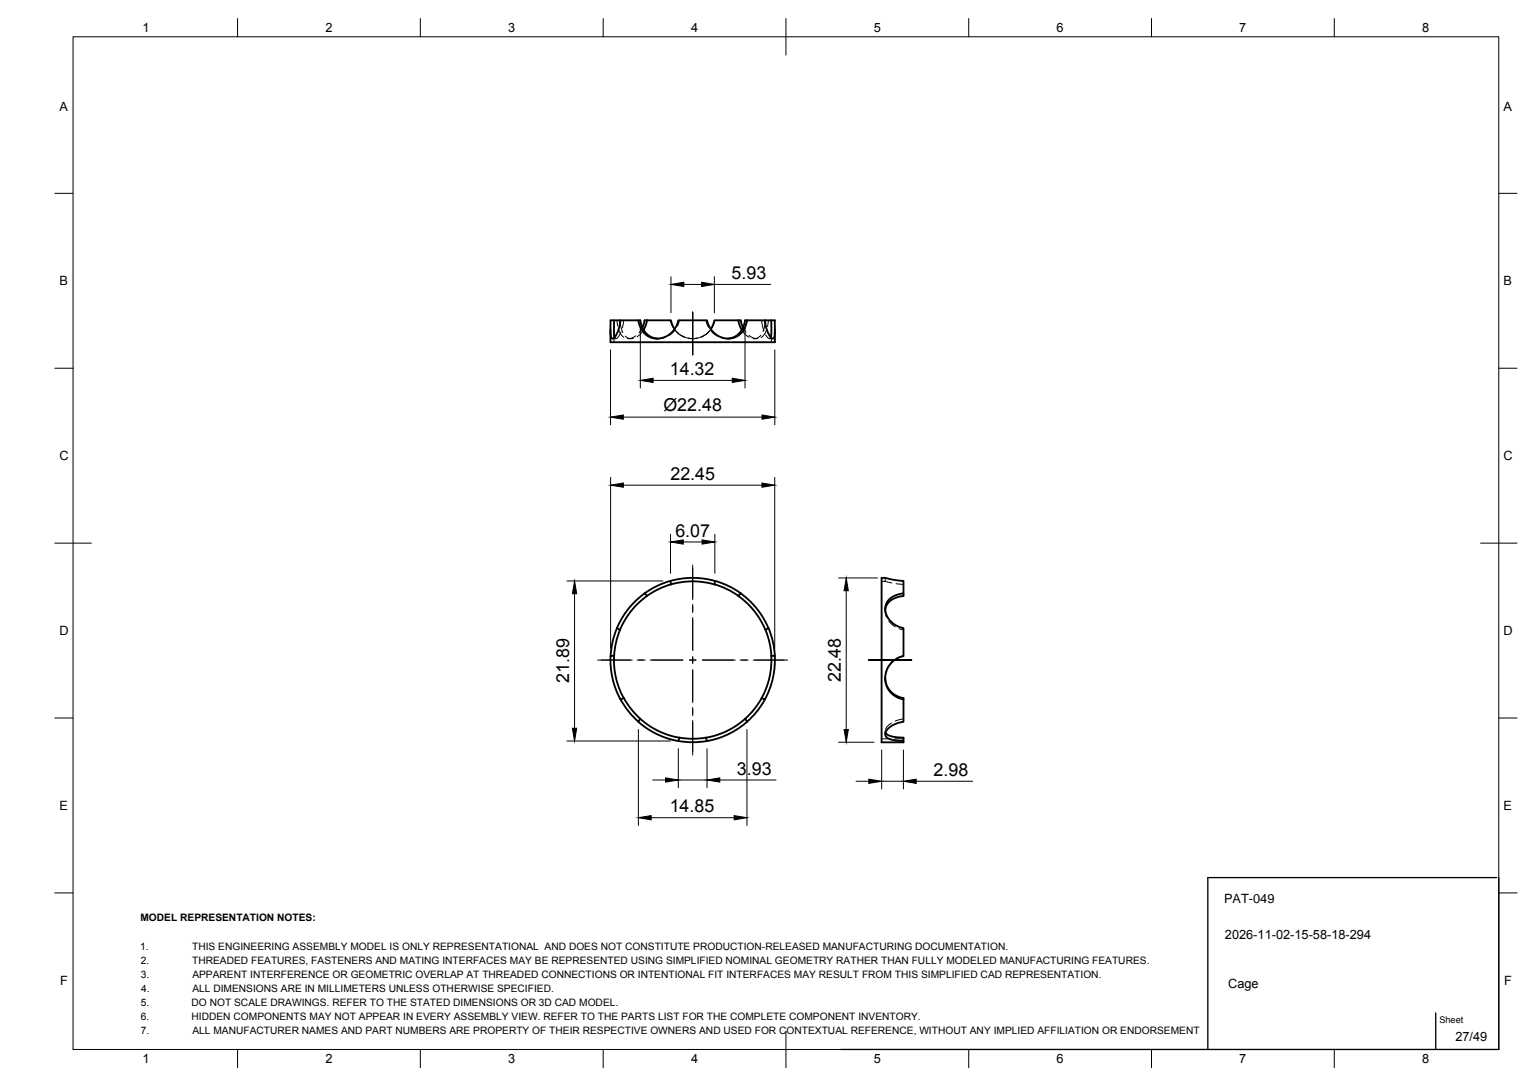
ISO-10303-21;
HEADER;
/* Generated by software containing ST-Developer
 * from STEP Tools, Inc. (www.steptools.com) 
 */

FILE_DESCRIPTION(
/* description */ ('Hand drill press frame (manual)'),
/* implementation_level */ '2;1');

FILE_NAME(
/* name */ 'Cage.step',
/* time_stamp */ '2026-10-28T03:25:28-07:00',
/* author */ (''),
/* organization */ (''),
/* preprocessor_version */ 'ST-DEVELOPER v20.2',
/* originating_system */ 'Autodesk Translation Framework v15.17.0.0',
/* authorisation */ '');

FILE_SCHEMA (('AUTOMOTIVE_DESIGN { 1 0 10303 214 3 1 1 }'));
ENDSEC;

DATA;
#10=MECHANICAL_DESIGN_GEOMETRIC_PRESENTATION_REPRESENTATION('',(#645),#33299);
#464=SPHERICAL_SURFACE('',#13660,0.309556);
#465=SPHERICAL_SURFACE('',#13676,0.309556);
#466=SPHERICAL_SURFACE('',#13681,0.309556);
#467=SPHERICAL_SURFACE('',#13687,0.309556);
#468=SPHERICAL_SURFACE('',#13692,0.309556);
#469=SPHERICAL_SURFACE('',#13697,0.309556);
#470=SPHERICAL_SURFACE('',#13705,0.309556);
#506=B_SPLINE_CURVE_WITH_KNOTS('',3,(#19268,#19269,#19270,#19271,#19272,
#19273,#19274,#19275,#19276,#19277,#19278,#19279,#19280,#19281,#19282,#19283,
#19284,#19285,#19286,#19287,#19288,#19289),.UNSPECIFIED.,.F.,.F.,(4,2,2,
2,2,2,2,2,2,2,4),(0.0591825211272536,0.157966726598481,0.236950089897721,
0.315933453196962,0.391576304923761,0.46721915665056,0.54286200837736,0.618504860104159,
0.697488223403399,0.77647158670264,0.875255792173867),.UNSPECIFIED.);
#507=B_SPLINE_CURVE_WITH_KNOTS('',3,(#19293,#19294,#19295,#19296,#19297,
#19298,#19299,#19300,#19301,#19302,#19303,#19304,#19305,#19306,#19307,#19308,
#19309,#19310,#19311,#19312,#19313,#19314),.UNSPECIFIED.,.F.,.F.,(4,2,2,
2,2,2,2,2,2,2,4),(0.0581119756758434,0.106553146291161,0.213106292582322,
0.30849933801665,0.386091982889075,0.4636846277615,0.541277272633925,0.61886991750635,
0.714262962940678,0.820816109231839,0.869257279847157),.UNSPECIFIED.);
#508=B_SPLINE_CURVE_WITH_KNOTS('',3,(#19320,#19321,#19322,#19323,#19324,
#19325,#19326,#19327,#19328,#19329,#19330,#19331,#19332,#19333,#19334,#19335,
#19336,#19337,#19338,#19339,#19340,#19341),.UNSPECIFIED.,.F.,.F.,(4,2,2,
2,2,2,2,2,2,2,4),(0.0581119756758434,0.106553146291161,0.213106292582322,
0.30849933801665,0.386091982889075,0.4636846277615,0.541277272633925,0.61886991750635,
0.714262962940679,0.820816109231839,0.869257279847157),.UNSPECIFIED.);
#509=B_SPLINE_CURVE_WITH_KNOTS('',3,(#19345,#19346,#19347,#19348,#19349,
#19350,#19351,#19352,#19353,#19354,#19355,#19356,#19357,#19358,#19359,#19360,
#19361,#19362,#19363,#19364,#19365,#19366),.UNSPECIFIED.,.F.,.F.,(4,2,2,
2,2,2,2,2,2,2,4),(0.0581119756758433,0.106553146291161,0.213106292582322,
0.308499338016649,0.386091982889075,0.4636846277615,0.541277272633925,0.61886991750635,
0.714262962940678,0.820816109231839,0.869257279847157),.UNSPECIFIED.);
#510=B_SPLINE_CURVE_WITH_KNOTS('',3,(#19375,#19376,#19377,#19378,#19379,
#19380,#19381,#19382,#19383,#19384,#19385,#19386,#19387,#19388,#19389,#19390,
#19391,#19392,#19393,#19394,#19395,#19396),.UNSPECIFIED.,.F.,.F.,(4,2,2,
2,2,2,2,2,2,2,4),(0.0581119756758433,0.106553146291161,0.213106292582322,
0.30849933801665,0.386091982889075,0.4636846277615,0.541277272633925,0.61886991750635,
0.714262962940678,0.820816109231839,0.869257279847157),.UNSPECIFIED.);
#511=B_SPLINE_CURVE_WITH_KNOTS('',3,(#19400,#19401,#19402,#19403,#19404,
#19405,#19406,#19407,#19408,#19409,#19410,#19411,#19412,#19413,#19414,#19415,
#19416,#19417,#19418,#19419,#19420,#19421),.UNSPECIFIED.,.F.,.F.,(4,2,2,
2,2,2,2,2,2,2,4),(0.0581119756758434,0.106553146291161,0.213106292582322,
0.30849933801665,0.386091982889075,0.4636846277615,0.541277272633925,0.61886991750635,
0.714262962940678,0.820816109231839,0.869257279847157),.UNSPECIFIED.);
#512=B_SPLINE_CURVE_WITH_KNOTS('',3,(#19425,#19426,#19427,#19428,#19429,
#19430,#19431,#19432,#19433,#19434,#19435,#19436,#19437,#19438,#19439,#19440,
#19441,#19442,#19443,#19444,#19445,#19446),.UNSPECIFIED.,.F.,.F.,(4,2,2,
2,2,2,2,2,2,2,4),(0.0581119756758434,0.106553146291161,0.213106292582322,
0.30849933801665,0.386091982889075,0.4636846277615,0.541277272633925,0.61886991750635,
0.714262962940678,0.820816109231839,0.869257279847157),.UNSPECIFIED.);
#513=B_SPLINE_CURVE_WITH_KNOTS('',3,(#19450,#19451,#19452,#19453,#19454,
#19455,#19456,#19457,#19458,#19459,#19460,#19461,#19462,#19463,#19464,#19465,
#19466,#19467,#19468,#19469,#19470,#19471),.UNSPECIFIED.,.F.,.F.,(4,2,2,
2,2,2,2,2,2,2,4),(0.0581119756758433,0.106553146291161,0.213106292582322,
0.30849933801665,0.386091982889075,0.4636846277615,0.541277272633925,0.61886991750635,
0.714262962940678,0.820816109231839,0.869257279847157),.UNSPECIFIED.);
#514=B_SPLINE_CURVE_WITH_KNOTS('',3,(#19479,#19480,#19481,#19482,#19483,
#19484,#19485,#19486,#19487,#19488,#19489,#19490,#19491,#19492,#19493,#19494,
#19495,#19496,#19497,#19498,#19499,#19500),.UNSPECIFIED.,.F.,.F.,(4,2,2,
2,2,2,2,2,2,2,4),(0.0591825211272536,0.157966726598481,0.236950089897721,
0.315933453196962,0.391576304923761,0.467219156650561,0.54286200837736,
0.618504860104159,0.697488223403399,0.77647158670264,0.875255792173867),
 .UNSPECIFIED.);
#515=B_SPLINE_CURVE_WITH_KNOTS('',3,(#19508,#19509,#19510,#19511,#19512,
#19513,#19514,#19515,#19516,#19517,#19518,#19519,#19520,#19521,#19522,#19523,
#19524,#19525,#19526,#19527,#19528,#19529),.UNSPECIFIED.,.F.,.F.,(4,2,2,
2,2,2,2,2,2,2,4),(0.0591825211272536,0.157966726598481,0.236950089897722,
0.315933453196962,0.391576304923761,0.467219156650561,0.54286200837736,
0.618504860104159,0.697488223403399,0.77647158670264,0.875255792173867),
 .UNSPECIFIED.);
#516=B_SPLINE_CURVE_WITH_KNOTS('',3,(#19539,#19540,#19541,#19542,#19543,
#19544,#19545,#19546,#19547,#19548,#19549,#19550,#19551,#19552,#19553,#19554,
#19555,#19556,#19557,#19558,#19559,#19560),.UNSPECIFIED.,.F.,.F.,(4,2,2,
2,2,2,2,2,2,2,4),(0.0591825211272536,0.157966726598481,0.236950089897721,
0.315933453196962,0.391576304923761,0.46721915665056,0.54286200837736,0.618504860104159,
0.697488223403399,0.77647158670264,0.875255792173867),.UNSPECIFIED.);
#517=B_SPLINE_CURVE_WITH_KNOTS('',3,(#19568,#19569,#19570,#19571,#19572,
#19573,#19574,#19575,#19576,#19577,#19578,#19579,#19580,#19581,#19582,#19583,
#19584,#19585,#19586,#19587,#19588,#19589),.UNSPECIFIED.,.F.,.F.,(4,2,2,
2,2,2,2,2,2,2,4),(0.0591825211272536,0.157966726598481,0.236950089897721,
0.315933453196962,0.391576304923761,0.46721915665056,0.542862008377359,
0.618504860104159,0.697488223403399,0.776471586702639,0.875255792173867),
 .UNSPECIFIED.);
#518=B_SPLINE_CURVE_WITH_KNOTS('',3,(#19597,#19598,#19599,#19600,#19601,
#19602,#19603,#19604,#19605,#19606,#19607,#19608,#19609,#19610,#19611,#19612,
#19613,#19614,#19615,#19616,#19617,#19618),.UNSPECIFIED.,.F.,.F.,(4,2,2,
2,2,2,2,2,2,2,4),(0.0591825211272536,0.157966726598481,0.236950089897721,
0.315933453196962,0.391576304923761,0.46721915665056,0.54286200837736,0.618504860104159,
0.697488223403399,0.77647158670264,0.875255792173867),.UNSPECIFIED.);
#519=B_SPLINE_CURVE_WITH_KNOTS('',3,(#19627,#19628,#19629,#19630,#19631,
#19632,#19633,#19634,#19635,#19636,#19637,#19638,#19639,#19640,#19641,#19642,
#19643,#19644,#19645,#19646,#19647,#19648),.UNSPECIFIED.,.F.,.F.,(4,2,2,
2,2,2,2,2,2,2,4),(0.0591825211272536,0.157966726598481,0.236950089897721,
0.315933453196962,0.391576304923761,0.46721915665056,0.542862008377359,
0.618504860104159,0.697488223403399,0.776471586702639,0.875255792173867),
 .UNSPECIFIED.);
#549=SHAPE_REPRESENTATION_RELATIONSHIP('SRR','None',#33509,#594);
#594=ADVANCED_BREP_SHAPE_REPRESENTATION('',(#697),#33271);
#645=STYLED_ITEM('',(#33814),#697);
#697=MANIFOLD_SOLID_BREP('Continuous crown cage',#12663);
#840=FACE_BOUND('',#2404,.T.);
#1021=PLANE('',#13673);
#1022=PLANE('',#13678);
#1023=PLANE('',#13683);
#1024=PLANE('',#13689);
#1025=PLANE('',#13694);
#1026=PLANE('',#13703);
#1027=PLANE('',#13707);
#1028=PLANE('',#13708);
#1579=FACE_OUTER_BOUND('',#2388,.T.);
#1580=FACE_OUTER_BOUND('',#2389,.T.);
#1581=FACE_OUTER_BOUND('',#2390,.T.);
#1582=FACE_OUTER_BOUND('',#2391,.T.);
#1583=FACE_OUTER_BOUND('',#2392,.T.);
#1584=FACE_OUTER_BOUND('',#2393,.T.);
#1585=FACE_OUTER_BOUND('',#2394,.T.);
#1586=FACE_OUTER_BOUND('',#2395,.T.);
#1587=FACE_OUTER_BOUND('',#2396,.T.);
#1588=FACE_OUTER_BOUND('',#2397,.T.);
#1589=FACE_OUTER_BOUND('',#2398,.T.);
#1590=FACE_OUTER_BOUND('',#2399,.T.);
#1591=FACE_OUTER_BOUND('',#2400,.T.);
#1592=FACE_OUTER_BOUND('',#2401,.T.);
#1593=FACE_OUTER_BOUND('',#2402,.T.);
#1594=FACE_OUTER_BOUND('',#2403,.T.);
#1595=FACE_OUTER_BOUND('',#2405,.T.);
#2388=EDGE_LOOP('',(#9525,#9526,#9527,#9528));
#2389=EDGE_LOOP('',(#9529,#9530,#9531,#9532,#9533,#9534,#9535,#9536,#9537,
#9538,#9539,#9540,#9541,#9542,#9543,#9544,#9545,#9546));
#2390=EDGE_LOOP('',(#9547,#9548,#9549,#9550));
#2391=EDGE_LOOP('',(#9551,#9552,#9553,#9554));
#2392=EDGE_LOOP('',(#9555,#9556,#9557,#9558));
#2393=EDGE_LOOP('',(#9559,#9560,#9561,#9562));
#2394=EDGE_LOOP('',(#9563,#9564,#9565,#9566,#9567,#9568));
#2395=EDGE_LOOP('',(#9569,#9570,#9571,#9572));
#2396=EDGE_LOOP('',(#9573,#9574,#9575,#9576));
#2397=EDGE_LOOP('',(#9577,#9578,#9579,#9580));
#2398=EDGE_LOOP('',(#9581,#9582,#9583,#9584));
#2399=EDGE_LOOP('',(#9585,#9586,#9587,#9588));
#2400=EDGE_LOOP('',(#9589,#9590,#9591,#9592,#9593,#9594,#9595,#9596,#9597,
#9598,#9599,#9600,#9601,#9602,#9603,#9604,#9605,#9606));
#2401=EDGE_LOOP('',(#9607,#9608,#9609,#9610));
#2402=EDGE_LOOP('',(#9611,#9612,#9613,#9614));
#2403=EDGE_LOOP('',(#9615));
#2404=EDGE_LOOP('',(#9616));
#2405=EDGE_LOOP('',(#9617,#9618,#9619,#9620));
#3213=LINE('',#19370,#4378);
#3214=LINE('',#19623,#4379);
#4378=VECTOR('',#15654,1.123812);
#4379=VECTOR('',#15723,1.076188);
#5422=CIRCLE('',#13661,0.303778037777585);
#5423=CIRCLE('',#13662,0.303778037777585);
#5424=CIRCLE('',#13664,1.123812);
#5425=CIRCLE('',#13665,1.123812);
#5426=CIRCLE('',#13666,1.123812);
#5427=CIRCLE('',#13667,1.123812);
#5428=CIRCLE('',#13668,1.123812);
#5429=CIRCLE('',#13669,1.123812);
#5430=CIRCLE('',#13670,1.123812);
#5431=CIRCLE('',#13671,1.123812);
#5432=CIRCLE('',#13672,1.123812);
#5433=CIRCLE('',#13674,1.076188);
#5434=CIRCLE('',#13675,0.303778037777585);
#5435=CIRCLE('',#13677,0.303778037777585);
#5436=CIRCLE('',#13679,1.076188);
#5437=CIRCLE('',#13680,0.303778037777585);
#5438=CIRCLE('',#13682,0.303778037777585);
#5439=CIRCLE('',#13684,1.076188);
#5440=CIRCLE('',#13685,1.076188);
#5441=CIRCLE('',#13686,0.303778037777585);
#5442=CIRCLE('',#13688,0.303778037777585);
#5443=CIRCLE('',#13690,1.076188);
#5444=CIRCLE('',#13691,0.303778037777585);
#5445=CIRCLE('',#13693,0.303778037777585);
#5446=CIRCLE('',#13695,1.076188);
#5447=CIRCLE('',#13696,0.303778037777585);
#5448=CIRCLE('',#13698,0.303778037777585);
#5449=CIRCLE('',#13700,1.076188);
#5450=CIRCLE('',#13701,1.076188);
#5451=CIRCLE('',#13702,1.076188);
#5452=CIRCLE('',#13704,0.303778037777585);
#5453=CIRCLE('',#13706,0.303778037777585);
#5989=VERTEX_POINT('',#19266);
#5990=VERTEX_POINT('',#19267);
#5991=VERTEX_POINT('',#19290);
#5992=VERTEX_POINT('',#19292);
#5993=VERTEX_POINT('',#19317);
#5994=VERTEX_POINT('',#19319);
#5995=VERTEX_POINT('',#19342);
#5996=VERTEX_POINT('',#19344);
#5997=VERTEX_POINT('',#19367);
#5998=VERTEX_POINT('',#19369);
#5999=VERTEX_POINT('',#19372);
#6000=VERTEX_POINT('',#19374);
#6001=VERTEX_POINT('',#19397);
#6002=VERTEX_POINT('',#19399);
#6003=VERTEX_POINT('',#19422);
#6004=VERTEX_POINT('',#19424);
#6005=VERTEX_POINT('',#19447);
#6006=VERTEX_POINT('',#19449);
#6007=VERTEX_POINT('',#19474);
#6008=VERTEX_POINT('',#19478);
#6009=VERTEX_POINT('',#19503);
#6010=VERTEX_POINT('',#19507);
#6011=VERTEX_POINT('',#19532);
#6012=VERTEX_POINT('',#19534);
#6013=VERTEX_POINT('',#19538);
#6014=VERTEX_POINT('',#19563);
#6015=VERTEX_POINT('',#19567);
#6016=VERTEX_POINT('',#19592);
#6017=VERTEX_POINT('',#19596);
#6018=VERTEX_POINT('',#19621);
#6019=VERTEX_POINT('',#19624);
#6020=VERTEX_POINT('',#19626);
#7291=EDGE_CURVE('',#5989,#5990,#506,.T.);
#7292=EDGE_CURVE('',#5991,#5989,#5422,.T.);
#7293=EDGE_CURVE('',#5992,#5991,#507,.T.);
#7294=EDGE_CURVE('',#5990,#5992,#5423,.T.);
#7295=EDGE_CURVE('',#5993,#5991,#5424,.T.);
#7296=EDGE_CURVE('',#5993,#5994,#508,.T.);
#7297=EDGE_CURVE('',#5995,#5994,#5425,.T.);
#7298=EDGE_CURVE('',#5995,#5996,#509,.T.);
#7299=EDGE_CURVE('',#5997,#5996,#5426,.T.);
#7300=EDGE_CURVE('',#5997,#5998,#3213,.T.);
#7301=EDGE_CURVE('',#5998,#5998,#5427,.T.);
#7302=EDGE_CURVE('',#5999,#5997,#5428,.T.);
#7303=EDGE_CURVE('',#5999,#6000,#510,.T.);
#7304=EDGE_CURVE('',#6001,#6000,#5429,.T.);
#7305=EDGE_CURVE('',#6001,#6002,#511,.T.);
#7306=EDGE_CURVE('',#6003,#6002,#5430,.T.);
#7307=EDGE_CURVE('',#6003,#6004,#512,.T.);
#7308=EDGE_CURVE('',#6005,#6004,#5431,.T.);
#7309=EDGE_CURVE('',#6005,#6006,#513,.T.);
#7310=EDGE_CURVE('',#5992,#6006,#5432,.T.);
#7311=EDGE_CURVE('',#5989,#6007,#5433,.T.);
#7312=EDGE_CURVE('',#6007,#5993,#5434,.T.);
#7313=EDGE_CURVE('',#6008,#6007,#514,.T.);
#7314=EDGE_CURVE('',#5994,#6008,#5435,.T.);
#7315=EDGE_CURVE('',#6008,#6009,#5436,.T.);
#7316=EDGE_CURVE('',#6009,#5995,#5437,.T.);
#7317=EDGE_CURVE('',#6010,#6009,#515,.T.);
#7318=EDGE_CURVE('',#5996,#6010,#5438,.T.);
#7319=EDGE_CURVE('',#6010,#6011,#5439,.T.);
#7320=EDGE_CURVE('',#6011,#6012,#5440,.T.);
#7321=EDGE_CURVE('',#6012,#5999,#5441,.T.);
#7322=EDGE_CURVE('',#6013,#6012,#516,.T.);
#7323=EDGE_CURVE('',#6000,#6013,#5442,.T.);
#7324=EDGE_CURVE('',#6013,#6014,#5443,.T.);
#7325=EDGE_CURVE('',#6014,#6001,#5444,.T.);
#7326=EDGE_CURVE('',#6015,#6014,#517,.T.);
#7327=EDGE_CURVE('',#6002,#6015,#5445,.T.);
#7328=EDGE_CURVE('',#6015,#6016,#5446,.T.);
#7329=EDGE_CURVE('',#6016,#6003,#5447,.T.);
#7330=EDGE_CURVE('',#6017,#6016,#518,.T.);
#7331=EDGE_CURVE('',#6004,#6017,#5448,.T.);
#7332=EDGE_CURVE('',#6018,#6018,#5449,.T.);
#7333=EDGE_CURVE('',#6018,#6011,#3214,.T.);
#7334=EDGE_CURVE('',#6019,#5990,#5450,.T.);
#7335=EDGE_CURVE('',#6019,#6020,#519,.T.);
#7336=EDGE_CURVE('',#6017,#6020,#5451,.T.);
#7337=EDGE_CURVE('',#6006,#6019,#5452,.T.);
#7338=EDGE_CURVE('',#6020,#6005,#5453,.T.);
#9525=ORIENTED_EDGE('',*,*,#7291,.F.);
#9526=ORIENTED_EDGE('',*,*,#7292,.F.);
#9527=ORIENTED_EDGE('',*,*,#7293,.F.);
#9528=ORIENTED_EDGE('',*,*,#7294,.F.);
#9529=ORIENTED_EDGE('',*,*,#7293,.T.);
#9530=ORIENTED_EDGE('',*,*,#7295,.F.);
#9531=ORIENTED_EDGE('',*,*,#7296,.T.);
#9532=ORIENTED_EDGE('',*,*,#7297,.F.);
#9533=ORIENTED_EDGE('',*,*,#7298,.T.);
#9534=ORIENTED_EDGE('',*,*,#7299,.F.);
#9535=ORIENTED_EDGE('',*,*,#7300,.T.);
#9536=ORIENTED_EDGE('',*,*,#7301,.F.);
#9537=ORIENTED_EDGE('',*,*,#7300,.F.);
#9538=ORIENTED_EDGE('',*,*,#7302,.F.);
#9539=ORIENTED_EDGE('',*,*,#7303,.T.);
#9540=ORIENTED_EDGE('',*,*,#7304,.F.);
#9541=ORIENTED_EDGE('',*,*,#7305,.T.);
#9542=ORIENTED_EDGE('',*,*,#7306,.F.);
#9543=ORIENTED_EDGE('',*,*,#7307,.T.);
#9544=ORIENTED_EDGE('',*,*,#7308,.F.);
#9545=ORIENTED_EDGE('',*,*,#7309,.T.);
#9546=ORIENTED_EDGE('',*,*,#7310,.F.);
#9547=ORIENTED_EDGE('',*,*,#7292,.T.);
#9548=ORIENTED_EDGE('',*,*,#7311,.T.);
#9549=ORIENTED_EDGE('',*,*,#7312,.T.);
#9550=ORIENTED_EDGE('',*,*,#7295,.T.);
#9551=ORIENTED_EDGE('',*,*,#7313,.F.);
#9552=ORIENTED_EDGE('',*,*,#7314,.F.);
#9553=ORIENTED_EDGE('',*,*,#7296,.F.);
#9554=ORIENTED_EDGE('',*,*,#7312,.F.);
#9555=ORIENTED_EDGE('',*,*,#7314,.T.);
#9556=ORIENTED_EDGE('',*,*,#7315,.T.);
#9557=ORIENTED_EDGE('',*,*,#7316,.T.);
#9558=ORIENTED_EDGE('',*,*,#7297,.T.);
#9559=ORIENTED_EDGE('',*,*,#7317,.F.);
#9560=ORIENTED_EDGE('',*,*,#7318,.F.);
#9561=ORIENTED_EDGE('',*,*,#7298,.F.);
#9562=ORIENTED_EDGE('',*,*,#7316,.F.);
#9563=ORIENTED_EDGE('',*,*,#7318,.T.);
#9564=ORIENTED_EDGE('',*,*,#7319,.T.);
#9565=ORIENTED_EDGE('',*,*,#7320,.T.);
#9566=ORIENTED_EDGE('',*,*,#7321,.T.);
#9567=ORIENTED_EDGE('',*,*,#7302,.T.);
#9568=ORIENTED_EDGE('',*,*,#7299,.T.);
#9569=ORIENTED_EDGE('',*,*,#7322,.F.);
#9570=ORIENTED_EDGE('',*,*,#7323,.F.);
#9571=ORIENTED_EDGE('',*,*,#7303,.F.);
#9572=ORIENTED_EDGE('',*,*,#7321,.F.);
#9573=ORIENTED_EDGE('',*,*,#7323,.T.);
#9574=ORIENTED_EDGE('',*,*,#7324,.T.);
#9575=ORIENTED_EDGE('',*,*,#7325,.T.);
#9576=ORIENTED_EDGE('',*,*,#7304,.T.);
#9577=ORIENTED_EDGE('',*,*,#7326,.F.);
#9578=ORIENTED_EDGE('',*,*,#7327,.F.);
#9579=ORIENTED_EDGE('',*,*,#7305,.F.);
#9580=ORIENTED_EDGE('',*,*,#7325,.F.);
#9581=ORIENTED_EDGE('',*,*,#7327,.T.);
#9582=ORIENTED_EDGE('',*,*,#7328,.T.);
#9583=ORIENTED_EDGE('',*,*,#7329,.T.);
#9584=ORIENTED_EDGE('',*,*,#7306,.T.);
#9585=ORIENTED_EDGE('',*,*,#7307,.F.);
#9586=ORIENTED_EDGE('',*,*,#7329,.F.);
#9587=ORIENTED_EDGE('',*,*,#7330,.F.);
#9588=ORIENTED_EDGE('',*,*,#7331,.F.);
#9589=ORIENTED_EDGE('',*,*,#7332,.F.);
#9590=ORIENTED_EDGE('',*,*,#7333,.T.);
#9591=ORIENTED_EDGE('',*,*,#7319,.F.);
#9592=ORIENTED_EDGE('',*,*,#7317,.T.);
#9593=ORIENTED_EDGE('',*,*,#7315,.F.);
#9594=ORIENTED_EDGE('',*,*,#7313,.T.);
#9595=ORIENTED_EDGE('',*,*,#7311,.F.);
#9596=ORIENTED_EDGE('',*,*,#7291,.T.);
#9597=ORIENTED_EDGE('',*,*,#7334,.F.);
#9598=ORIENTED_EDGE('',*,*,#7335,.T.);
#9599=ORIENTED_EDGE('',*,*,#7336,.F.);
#9600=ORIENTED_EDGE('',*,*,#7330,.T.);
#9601=ORIENTED_EDGE('',*,*,#7328,.F.);
#9602=ORIENTED_EDGE('',*,*,#7326,.T.);
#9603=ORIENTED_EDGE('',*,*,#7324,.F.);
#9604=ORIENTED_EDGE('',*,*,#7322,.T.);
#9605=ORIENTED_EDGE('',*,*,#7320,.F.);
#9606=ORIENTED_EDGE('',*,*,#7333,.F.);
#9607=ORIENTED_EDGE('',*,*,#7294,.T.);
#9608=ORIENTED_EDGE('',*,*,#7310,.T.);
#9609=ORIENTED_EDGE('',*,*,#7337,.T.);
#9610=ORIENTED_EDGE('',*,*,#7334,.T.);
#9611=ORIENTED_EDGE('',*,*,#7309,.F.);
#9612=ORIENTED_EDGE('',*,*,#7338,.F.);
#9613=ORIENTED_EDGE('',*,*,#7335,.F.);
#9614=ORIENTED_EDGE('',*,*,#7337,.F.);
#9615=ORIENTED_EDGE('',*,*,#7301,.T.);
#9616=ORIENTED_EDGE('',*,*,#7332,.T.);
#9617=ORIENTED_EDGE('',*,*,#7331,.T.);
#9618=ORIENTED_EDGE('',*,*,#7336,.T.);
#9619=ORIENTED_EDGE('',*,*,#7338,.T.);
#9620=ORIENTED_EDGE('',*,*,#7308,.T.);
#11877=CYLINDRICAL_SURFACE('',#13663,1.123812);
#11878=CYLINDRICAL_SURFACE('',#13699,1.076188);
#12188=ADVANCED_FACE('',(#1579),#464,.F.);
#12189=ADVANCED_FACE('',(#1580),#11877,.T.);
#12190=ADVANCED_FACE('',(#1581),#1021,.T.);
#12191=ADVANCED_FACE('',(#1582),#465,.F.);
#12192=ADVANCED_FACE('',(#1583),#1022,.T.);
#12193=ADVANCED_FACE('',(#1584),#466,.F.);
#12194=ADVANCED_FACE('',(#1585),#1023,.T.);
#12195=ADVANCED_FACE('',(#1586),#467,.F.);
#12196=ADVANCED_FACE('',(#1587),#1024,.T.);
#12197=ADVANCED_FACE('',(#1588),#468,.F.);
#12198=ADVANCED_FACE('',(#1589),#1025,.T.);
#12199=ADVANCED_FACE('',(#1590),#469,.F.);
#12200=ADVANCED_FACE('',(#1591),#11878,.F.);
#12201=ADVANCED_FACE('',(#1592),#1026,.T.);
#12202=ADVANCED_FACE('',(#1593),#470,.F.);
#12203=ADVANCED_FACE('',(#1594,#840),#1027,.T.);
#12204=ADVANCED_FACE('',(#1595),#1028,.T.);
#12663=CLOSED_SHELL('',(#12188,#12189,#12190,#12191,#12192,#12193,#12194,
#12195,#12196,#12197,#12198,#12199,#12200,#12201,#12202,#12203,#12204));
#13659=AXIS2_PLACEMENT_3D('',#19264,#15638,#15639);
#13660=AXIS2_PLACEMENT_3D('',#19265,#15640,#15641);
#13661=AXIS2_PLACEMENT_3D('',#19291,#15642,#15643);
#13662=AXIS2_PLACEMENT_3D('',#19315,#15644,#15645);
#13663=AXIS2_PLACEMENT_3D('',#19316,#15646,#15647);
#13664=AXIS2_PLACEMENT_3D('',#19318,#15648,#15649);
#13665=AXIS2_PLACEMENT_3D('',#19343,#15650,#15651);
#13666=AXIS2_PLACEMENT_3D('',#19368,#15652,#15653);
#13667=AXIS2_PLACEMENT_3D('',#19371,#15655,#15656);
#13668=AXIS2_PLACEMENT_3D('',#19373,#15657,#15658);
#13669=AXIS2_PLACEMENT_3D('',#19398,#15659,#15660);
#13670=AXIS2_PLACEMENT_3D('',#19423,#15661,#15662);
#13671=AXIS2_PLACEMENT_3D('',#19448,#15663,#15664);
#13672=AXIS2_PLACEMENT_3D('',#19472,#15665,#15666);
#13673=AXIS2_PLACEMENT_3D('',#19473,#15667,#15668);
#13674=AXIS2_PLACEMENT_3D('',#19475,#15669,#15670);
#13675=AXIS2_PLACEMENT_3D('',#19476,#15671,#15672);
#13676=AXIS2_PLACEMENT_3D('',#19477,#15673,#15674);
#13677=AXIS2_PLACEMENT_3D('',#19501,#15675,#15676);
#13678=AXIS2_PLACEMENT_3D('',#19502,#15677,#15678);
#13679=AXIS2_PLACEMENT_3D('',#19504,#15679,#15680);
#13680=AXIS2_PLACEMENT_3D('',#19505,#15681,#15682);
#13681=AXIS2_PLACEMENT_3D('',#19506,#15683,#15684);
#13682=AXIS2_PLACEMENT_3D('',#19530,#15685,#15686);
#13683=AXIS2_PLACEMENT_3D('',#19531,#15687,#15688);
#13684=AXIS2_PLACEMENT_3D('',#19533,#15689,#15690);
#13685=AXIS2_PLACEMENT_3D('',#19535,#15691,#15692);
#13686=AXIS2_PLACEMENT_3D('',#19536,#15693,#15694);
#13687=AXIS2_PLACEMENT_3D('',#19537,#15695,#15696);
#13688=AXIS2_PLACEMENT_3D('',#19561,#15697,#15698);
#13689=AXIS2_PLACEMENT_3D('',#19562,#15699,#15700);
#13690=AXIS2_PLACEMENT_3D('',#19564,#15701,#15702);
#13691=AXIS2_PLACEMENT_3D('',#19565,#15703,#15704);
#13692=AXIS2_PLACEMENT_3D('',#19566,#15705,#15706);
#13693=AXIS2_PLACEMENT_3D('',#19590,#15707,#15708);
#13694=AXIS2_PLACEMENT_3D('',#19591,#15709,#15710);
#13695=AXIS2_PLACEMENT_3D('',#19593,#15711,#15712);
#13696=AXIS2_PLACEMENT_3D('',#19594,#15713,#15714);
#13697=AXIS2_PLACEMENT_3D('',#19595,#15715,#15716);
#13698=AXIS2_PLACEMENT_3D('',#19619,#15717,#15718);
#13699=AXIS2_PLACEMENT_3D('',#19620,#15719,#15720);
#13700=AXIS2_PLACEMENT_3D('',#19622,#15721,#15722);
#13701=AXIS2_PLACEMENT_3D('',#19625,#15724,#15725);
#13702=AXIS2_PLACEMENT_3D('',#19649,#15726,#15727);
#13703=AXIS2_PLACEMENT_3D('',#19650,#15728,#15729);
#13704=AXIS2_PLACEMENT_3D('',#19651,#15730,#15731);
#13705=AXIS2_PLACEMENT_3D('',#19652,#15732,#15733);
#13706=AXIS2_PLACEMENT_3D('',#19653,#15734,#15735);
#13707=AXIS2_PLACEMENT_3D('',#19654,#15736,#15737);
#13708=AXIS2_PLACEMENT_3D('',#19655,#15738,#15739);
#15638=DIRECTION('axis',(0.,0.,1.));
#15639=DIRECTION('refdir',(1.,0.,0.));
#15640=DIRECTION('center_axis',(0.,0.,1.));
#15641=DIRECTION('ref_axis',(1.,0.,0.));
#15642=DIRECTION('center_axis',(0.,-1.,0.));
#15643=DIRECTION('ref_axis',(0.,0.,-1.));
#15644=DIRECTION('center_axis',(0.,-1.,0.));
#15645=DIRECTION('ref_axis',(0.,0.,-1.));
#15646=DIRECTION('center_axis',(0.,1.,0.));
#15647=DIRECTION('ref_axis',(1.,0.,0.));
#15648=DIRECTION('center_axis',(0.,1.,0.));
#15649=DIRECTION('ref_axis',(1.,0.,0.));
#15650=DIRECTION('center_axis',(0.,1.,0.));
#15651=DIRECTION('ref_axis',(1.,0.,0.));
#15652=DIRECTION('center_axis',(0.,1.,0.));
#15653=DIRECTION('ref_axis',(1.,0.,0.));
#15654=DIRECTION('',(0.,-1.,0.));
#15655=DIRECTION('center_axis',(0.,-1.,0.));
#15656=DIRECTION('ref_axis',(1.,0.,0.));
#15657=DIRECTION('center_axis',(0.,1.,0.));
#15658=DIRECTION('ref_axis',(1.,0.,0.));
#15659=DIRECTION('center_axis',(0.,1.,0.));
#15660=DIRECTION('ref_axis',(1.,0.,0.));
#15661=DIRECTION('center_axis',(0.,1.,0.));
#15662=DIRECTION('ref_axis',(1.,0.,0.));
#15663=DIRECTION('center_axis',(0.,1.,0.));
#15664=DIRECTION('ref_axis',(1.,0.,0.));
#15665=DIRECTION('center_axis',(0.,1.,0.));
#15666=DIRECTION('ref_axis',(1.,0.,0.));
#15667=DIRECTION('center_axis',(0.,1.,0.));
#15668=DIRECTION('ref_axis',(1.,0.,0.));
#15669=DIRECTION('center_axis',(0.,-1.,0.));
#15670=DIRECTION('ref_axis',(1.,0.,0.));
#15671=DIRECTION('center_axis',(0.,-1.,0.));
#15672=DIRECTION('ref_axis',(0.,0.,-1.));
#15673=DIRECTION('center_axis',(8.96625347776458E-17,0.,1.));
#15674=DIRECTION('ref_axis',(1.,0.,0.));
#15675=DIRECTION('center_axis',(0.,-1.,0.));
#15676=DIRECTION('ref_axis',(0.,0.,-1.));
#15677=DIRECTION('center_axis',(0.,1.,0.));
#15678=DIRECTION('ref_axis',(1.,0.,0.));
#15679=DIRECTION('center_axis',(0.,-1.,0.));
#15680=DIRECTION('ref_axis',(1.,0.,0.));
#15681=DIRECTION('center_axis',(0.,-1.,0.));
#15682=DIRECTION('ref_axis',(0.,0.,-1.));
#15683=DIRECTION('center_axis',(0.,0.,1.));
#15684=DIRECTION('ref_axis',(1.,0.,0.));
#15685=DIRECTION('center_axis',(0.,-1.,0.));
#15686=DIRECTION('ref_axis',(0.,0.,-1.));
#15687=DIRECTION('center_axis',(0.,1.,0.));
#15688=DIRECTION('ref_axis',(1.,0.,0.));
#15689=DIRECTION('center_axis',(0.,-1.,0.));
#15690=DIRECTION('ref_axis',(1.,0.,0.));
#15691=DIRECTION('center_axis',(0.,-1.,0.));
#15692=DIRECTION('ref_axis',(1.,0.,0.));
#15693=DIRECTION('center_axis',(0.,-1.,0.));
#15694=DIRECTION('ref_axis',(0.,0.,-1.));
#15695=DIRECTION('center_axis',(0.,0.,1.));
#15696=DIRECTION('ref_axis',(1.,0.,0.));
#15697=DIRECTION('center_axis',(0.,-1.,0.));
#15698=DIRECTION('ref_axis',(0.,0.,-1.));
#15699=DIRECTION('center_axis',(0.,1.,0.));
#15700=DIRECTION('ref_axis',(1.,0.,0.));
#15701=DIRECTION('center_axis',(0.,-1.,0.));
#15702=DIRECTION('ref_axis',(1.,0.,0.));
#15703=DIRECTION('center_axis',(0.,-1.,0.));
#15704=DIRECTION('ref_axis',(0.,0.,-1.));
#15705=DIRECTION('center_axis',(8.96625347776458E-17,0.,1.));
#15706=DIRECTION('ref_axis',(1.,0.,0.));
#15707=DIRECTION('center_axis',(0.,-1.,0.));
#15708=DIRECTION('ref_axis',(0.,0.,-1.));
#15709=DIRECTION('center_axis',(0.,1.,0.));
#15710=DIRECTION('ref_axis',(1.,0.,0.));
#15711=DIRECTION('center_axis',(0.,-1.,0.));
#15712=DIRECTION('ref_axis',(1.,0.,0.));
#15713=DIRECTION('center_axis',(0.,-1.,0.));
#15714=DIRECTION('ref_axis',(0.,0.,-1.));
#15715=DIRECTION('center_axis',(0.,0.,1.));
#15716=DIRECTION('ref_axis',(1.,0.,0.));
#15717=DIRECTION('center_axis',(0.,-1.,0.));
#15718=DIRECTION('ref_axis',(0.,0.,-1.));
#15719=DIRECTION('center_axis',(0.,1.,0.));
#15720=DIRECTION('ref_axis',(1.,0.,0.));
#15721=DIRECTION('center_axis',(0.,1.,0.));
#15722=DIRECTION('ref_axis',(1.,0.,0.));
#15723=DIRECTION('',(0.,1.,0.));
#15724=DIRECTION('center_axis',(0.,-1.,0.));
#15725=DIRECTION('ref_axis',(1.,0.,0.));
#15726=DIRECTION('center_axis',(0.,-1.,0.));
#15727=DIRECTION('ref_axis',(1.,0.,0.));
#15728=DIRECTION('center_axis',(0.,1.,0.));
#15729=DIRECTION('ref_axis',(1.,0.,0.));
#15730=DIRECTION('center_axis',(0.,-1.,0.));
#15731=DIRECTION('ref_axis',(0.,0.,-1.));
#15732=DIRECTION('center_axis',(0.,0.,1.));
#15733=DIRECTION('ref_axis',(1.,0.,0.));
#15734=DIRECTION('center_axis',(0.,-1.,0.));
#15735=DIRECTION('ref_axis',(0.,0.,-1.));
#15736=DIRECTION('center_axis',(0.,-1.,0.));
#15737=DIRECTION('ref_axis',(-1.,0.,0.));
#15738=DIRECTION('center_axis',(0.,1.,0.));
#15739=DIRECTION('ref_axis',(1.,0.,0.));
#19264=CARTESIAN_POINT('',(0.,0.,0.));
#19265=CARTESIAN_POINT('Origin',(0.685838782044607,0.,0.860014630714833));
#19266=CARTESIAN_POINT('',(0.413083465285518,-0.05953,0.993751811093549));
#19267=CARTESIAN_POINT('',(0.876916659919095,-0.05953,0.623857181492959));
#19268=CARTESIAN_POINT('Ctrl Pts',(0.413083465285518,-0.05953,0.993751811093549));
#19269=CARTESIAN_POINT('Ctrl Pts',(0.419070565453383,-0.0925528133349865,
0.991263089003441));
#19270=CARTESIAN_POINT('Ctrl Pts',(0.430199341854858,-0.124911173756694,
0.986608710139579));
#19271=CARTESIAN_POINT('Ctrl Pts',(0.457978755888596,-0.177924977804098,
0.973971221090534));
#19272=CARTESIAN_POINT('Ctrl Pts',(0.473077587363685,-0.199697230012983,
0.966820759530997));
#19273=CARTESIAN_POINT('Ctrl Pts',(0.507057380724533,-0.237895043532788,
0.949440676105255));
#19274=CARTESIAN_POINT('Ctrl Pts',(0.525933334162555,-0.254319232363049,
0.939198248544428));
#19275=CARTESIAN_POINT('Ctrl Pts',(0.564362943424238,-0.28018331644634,
0.916597376014514));
#19276=CARTESIAN_POINT('Ctrl Pts',(0.585840553788742,-0.29104845371857,
0.903141581680914));
#19277=CARTESIAN_POINT('Ctrl Pts',(0.629305439856167,-0.30527573347708,
0.873412008702649));
#19278=CARTESIAN_POINT('Ctrl Pts',(0.651278921914856,-0.308638795020976,
0.857118508332695));
#19279=CARTESIAN_POINT('Ctrl Pts',(0.690705563850638,-0.308638795020976,
0.825676810575914));
#19280=CARTESIAN_POINT('Ctrl Pts',(0.711480111898423,-0.30527573347708,
0.807879894508811));
#19281=CARTESIAN_POINT('Ctrl Pts',(0.750136149454208,-0.29104845371857,
0.772120216227122));
#19282=CARTESIAN_POINT('Ctrl Pts',(0.768033796848072,-0.28018331644634,
0.754175290318038));
#19283=CARTESIAN_POINT('Ctrl Pts',(0.798619410861634,-0.254319232363049,
0.721738358858166));
#19284=CARTESIAN_POINT('Ctrl Pts',(0.812805334167529,-0.237895043532788,
0.705614819529209));
#19285=CARTESIAN_POINT('Ctrl Pts',(0.837310877969633,-0.199697230012983,
0.676354402927683));
#19286=CARTESIAN_POINT('Ctrl Pts',(0.847641868610495,-0.177924977804098,
0.663225258065736));
#19287=CARTESIAN_POINT('Ctrl Pts',(0.866144010579847,-0.124911173756694,
0.638954437806245));
#19288=CARTESIAN_POINT('Ctrl Pts',(0.873158080166742,-0.0925528133349865,
0.62914037979579));
#19289=CARTESIAN_POINT('Ctrl Pts',(0.876916659919095,-0.05953,0.623857181492959));
#19290=CARTESIAN_POINT('',(0.437601487681057,-0.05953,1.03511272300331));
#19291=CARTESIAN_POINT('Origin',(0.685838782044607,-0.05953,0.860014630714833));
#19292=CARTESIAN_POINT('',(0.911784794170997,-0.05953,0.656964154625313));
#19293=CARTESIAN_POINT('Ctrl Pts',(0.911784794170998,-0.0595300000000001,
0.656964154625312));
#19294=CARTESIAN_POINT('Ctrl Pts',(0.909827729890942,-0.0762225747374255,
0.659680317203144));
#19295=CARTESIAN_POINT('Ctrl Pts',(0.907004864562642,-0.0928409665394228,
0.663576540841106));
#19296=CARTESIAN_POINT('Ctrl Pts',(0.895234408667242,-0.144299303100741,
0.679480524217551));
#19297=CARTESIAN_POINT('Ctrl Pts',(0.882797231409153,-0.177024326825049,
0.695831250979106));
#19298=CARTESIAN_POINT('Ctrl Pts',(0.854332839576145,-0.227269801620064,
0.73042219438957));
#19299=CARTESIAN_POINT('Ctrl Pts',(0.834863020612702,-0.251265615809407,
0.752807465209441));
#19300=CARTESIAN_POINT('Ctrl Pts',(0.800439809856111,-0.279889827963178,
0.789147407129766));
#19301=CARTESIAN_POINT('Ctrl Pts',(0.781998747691871,-0.290879136862659,
0.80756613568454));
#19302=CARTESIAN_POINT('Ctrl Pts',(0.742239891936898,-0.305251990234487,
0.844254137480382));
#19303=CARTESIAN_POINT('Ctrl Pts',(0.720906778729541,-0.308638795020976,
0.862505527716294));
#19304=CARTESIAN_POINT('Ctrl Pts',(0.680463863683392,-0.308638795020976,
0.894757676234429));
#19305=CARTESIAN_POINT('Ctrl Pts',(0.657923009631182,-0.305251990234488,
0.91149460735272));
#19306=CARTESIAN_POINT('Ctrl Pts',(0.613307674922609,-0.290879136862659,
0.942092777160053));
#19307=CARTESIAN_POINT('Ctrl Pts',(0.591247219971725,-0.279889827963178,
0.955972930713954));
#19308=CARTESIAN_POINT('Ctrl Pts',(0.548158511259202,-0.251265615809407,
0.981446681891443));
#19309=CARTESIAN_POINT('Ctrl Pts',(0.522002043615455,-0.227269801620063,
0.995447160474328));
#19310=CARTESIAN_POINT('Ctrl Pts',(0.481944444320713,-0.177024326825049,
1.01550068154148));
#19311=CARTESIAN_POINT('Ctrl Pts',(0.463236132117164,-0.14429930310074,
1.0239876538093));
#19312=CARTESIAN_POINT('Ctrl Pts',(0.445111721969657,-0.0928409665394226,
1.03192403056628));
#19313=CARTESIAN_POINT('Ctrl Pts',(0.440685038163619,-0.0762225747374254,
1.03380912944435));
#19314=CARTESIAN_POINT('Ctrl Pts',(0.437601487681056,-0.05953,1.03511272300331));
#19315=CARTESIAN_POINT('Origin',(0.685838782044607,-0.05953,0.860014630714833));
#19316=CARTESIAN_POINT('Origin',(0.,-0.208355,0.));
#19317=CARTESIAN_POINT('',(0.0548532617164168,-0.05953,1.12247250791415));
#19318=CARTESIAN_POINT('Origin',(0.,-0.05953,0.));
#19319=CARTESIAN_POINT('',(-0.536443649899848,-0.05953,0.987512846410683));
#19320=CARTESIAN_POINT('Ctrl Pts',(0.0548532617164173,-0.0595300000000001,
1.12247250791414));
#19321=CARTESIAN_POINT('Ctrl Pts',(0.05150947068137,-0.0762225747374254,
1.12263591311425));
#19322=CARTESIAN_POINT('Ctrl Pts',(0.0467032526342597,-0.0928409665394227,
1.12285816383385));
#19323=CARTESIAN_POINT('Ctrl Pts',(0.0269302585198975,-0.144299303100741,
1.12357162229597));
#19324=CARTESIAN_POINT('Ctrl Pts',(0.006392292392153,-0.177024326825049,
1.12404235695137));
#19325=CARTESIAN_POINT('Ctrl Pts',(-0.0383992541984087,-0.227269801620063,
1.12335509974011));
#19326=CARTESIAN_POINT('Ctrl Pts',(-0.0680399972366993,-0.251265615809407,
1.12208997038458));
#19327=CARTESIAN_POINT('Ctrl Pts',(-0.117914228755037,-0.279889827963178,
1.1178344036749));
#19328=CARTESIAN_POINT('Ctrl Pts',(-0.14381238480104,-0.290879136862659,
1.11490049012186));
#19329=CARTESIAN_POINT('Ctrl Pts',(-0.19728546073067,-0.305251990234488,
1.10669035995599));
#19330=CARTESIAN_POINT('Ctrl Pts',(-0.224855950742601,-0.308638795020976,
1.10139101611326));
#19331=CARTESIAN_POINT('Ctrl Pts',(-0.275287440920027,-0.308638795020976,
1.0898803575765));
#19332=CARTESIAN_POINT('Ctrl Pts',(-0.302426893214945,-0.305251990234488,
1.08269251410343));
#19333=CARTESIAN_POINT('Ctrl Pts',(-0.35416671187353,-0.290879136862659,
1.06688848765783));
#19334=CARTESIAN_POINT('Ctrl Pts',(-0.3787731215897,-0.279889827963178,
1.05829506364875));
#19335=CARTESIAN_POINT('Ctrl Pts',(-0.425554672694338,-0.251265615809407,
1.04048957871266));
#19336=CARTESIAN_POINT('Ctrl Pts',(-0.452808978448581,-0.227269801620063,
1.02876878445619));
#19337=CARTESIAN_POINT('Ctrl Pts',(-0.493462957200432,-0.177024326825049,
1.0099536580922));
#19338=CARTESIAN_POINT('Ctrl Pts',(-0.511762781179148,-0.14429930310074,
1.00061845128527));
#19339=CARTESIAN_POINT('Ctrl Pts',(-0.529268075276157,-0.0928409665394226,
0.991396466802468));
#19340=CARTESIAN_POINT('Ctrl Pts',(-0.533501897135713,-0.0762225747374254,
0.989110885965947));
#19341=CARTESIAN_POINT('Ctrl Pts',(-0.536443649899848,-0.0595300000000001,
0.987512846410683));
#19342=CARTESIAN_POINT('',(-0.843383895613249,-0.05953,0.742736168477219));
#19343=CARTESIAN_POINT('Origin',(0.,-0.05953,0.));
#19344=CARTESIAN_POINT('',(-1.10653577764992,-0.05953,0.196295654879792));
#19345=CARTESIAN_POINT('Ctrl Pts',(-0.843383895613249,-0.0595300000000001,
0.742736168477219));
#19346=CARTESIAN_POINT('Ctrl Pts',(-0.84559647055299,-0.0762225747374255,
0.740223768851062));
#19347=CARTESIAN_POINT('Ctrl Pts',(-0.848766861100456,-0.0928409665394227,
0.736604687327351));
#19348=CARTESIAN_POINT('Ctrl Pts',(-0.861652925570091,-0.144299303100741,
0.721590372101268));
#19349=CARTESIAN_POINT('Ctrl Pts',(-0.87482617317514,-0.177024326825049,
0.705826641853758));
#19350=CARTESIAN_POINT('Ctrl Pts',(-0.902215926359523,-0.227269801620063,
0.670378702718353));
#19351=CARTESIAN_POINT('Ctrl Pts',(-0.919707509403859,-0.251265615809407,
0.646415841396062));
#19352=CARTESIAN_POINT('Ctrl Pts',(-0.947476448101718,-0.279889827963178,
0.604769294586516));
#19353=CARTESIAN_POINT('Ctrl Pts',(-0.961329858300736,-0.290879136862659,
0.582692035672022));
#19354=CARTESIAN_POINT('Ctrl Pts',(-0.988250837578047,-0.305251990234488,
0.535766169015486));
#19355=CARTESIAN_POINT('Ctrl Pts',(-1.00129756308006,-0.308638795020976,
0.510906605094603));
#19356=CARTESIAN_POINT('Ctrl Pts',(-1.02374168767024,-0.308638795020976,
0.46430090015576));
#19357=CARTESIAN_POINT('Ctrl Pts',(-1.03504317708586,-0.305251990234488,
0.438600874831839));
#19358=CARTESIAN_POINT('Ctrl Pts',(-1.05494634094458,-0.290879136862659,
0.388295406390235));
#19359=CARTESIAN_POINT('Ctrl Pts',(-1.06356957703048,-0.279889827963178,
0.363699428370917));
#19360=CARTESIAN_POINT('Ctrl Pts',(-1.0788165083757,-0.251265615809407,
0.316022600643821));
#19361=CARTESIAN_POINT('Ctrl Pts',(-1.08664560412098,-0.227269801620063,
0.287406530683752));
#19362=CARTESIAN_POINT('Ctrl Pts',(-1.09728268713976,-0.177024326825049,
0.243890930799337));
#19363=CARTESIAN_POINT('Ctrl Pts',(-1.10139388218929,-0.144299303100741,
0.22376314604679));
#19364=CARTESIAN_POINT('Ctrl Pts',(-1.10509821673782,-0.0928409665394227,
0.204327142733961));
#19365=CARTESIAN_POINT('Ctrl Pts',(-1.10595102243643,-0.0762225747374254,
0.199591971170104));
#19366=CARTESIAN_POINT('Ctrl Pts',(-1.10653577764992,-0.0595300000000001,
0.196295654879792));
#19367=CARTESIAN_POINT('',(-1.123812,-0.05953,1.37627276864339E-16));
#19368=CARTESIAN_POINT('Origin',(0.,-0.05953,0.));
#19369=CARTESIAN_POINT('',(-1.123812,-0.35718,1.37627276864339E-16));
#19370=CARTESIAN_POINT('',(-1.123812,-0.208355,1.37627276864339E-16));
#19371=CARTESIAN_POINT('Origin',(0.,-0.35718,0.));
#19372=CARTESIAN_POINT('',(-1.10653577764992,-0.05953,-0.196295654879793));
#19373=CARTESIAN_POINT('Origin',(0.,-0.05953,0.));
#19374=CARTESIAN_POINT('',(-0.843383895613249,-0.05953,-0.742736168477219));
#19375=CARTESIAN_POINT('Ctrl Pts',(-1.10653577764992,-0.0595300000000001,
-0.196295654879792));
#19376=CARTESIAN_POINT('Ctrl Pts',(-1.10595102243643,-0.0762225747374255,
-0.199591971170104));
#19377=CARTESIAN_POINT('Ctrl Pts',(-1.10509821673782,-0.0928409665394228,
-0.204327142733962));
#19378=CARTESIAN_POINT('Ctrl Pts',(-1.10139388218929,-0.144299303100741,
-0.22376314604679));
#19379=CARTESIAN_POINT('Ctrl Pts',(-1.09728268713976,-0.177024326825049,
-0.243890930799338));
#19380=CARTESIAN_POINT('Ctrl Pts',(-1.08664560412098,-0.227269801620063,
-0.287406530683753));
#19381=CARTESIAN_POINT('Ctrl Pts',(-1.0788165083757,-0.251265615809407,
-0.316022600643821));
#19382=CARTESIAN_POINT('Ctrl Pts',(-1.06356957703048,-0.279889827963178,
-0.363699428370918));
#19383=CARTESIAN_POINT('Ctrl Pts',(-1.05494634094458,-0.290879136862659,
-0.388295406390235));
#19384=CARTESIAN_POINT('Ctrl Pts',(-1.03504317708586,-0.305251990234488,
-0.438600874831839));
#19385=CARTESIAN_POINT('Ctrl Pts',(-1.02374168767024,-0.308638795020976,
-0.46430090015576));
#19386=CARTESIAN_POINT('Ctrl Pts',(-1.00129756308006,-0.308638795020976,
-0.510906605094603));
#19387=CARTESIAN_POINT('Ctrl Pts',(-0.988250837578047,-0.305251990234488,
-0.535766169015486));
#19388=CARTESIAN_POINT('Ctrl Pts',(-0.961329858300736,-0.290879136862659,
-0.582692035672022));
#19389=CARTESIAN_POINT('Ctrl Pts',(-0.947476448101718,-0.279889827963178,
-0.604769294586516));
#19390=CARTESIAN_POINT('Ctrl Pts',(-0.919707509403859,-0.251265615809407,
-0.646415841396062));
#19391=CARTESIAN_POINT('Ctrl Pts',(-0.902215926359523,-0.227269801620064,
-0.670378702718353));
#19392=CARTESIAN_POINT('Ctrl Pts',(-0.87482617317514,-0.177024326825049,
-0.705826641853758));
#19393=CARTESIAN_POINT('Ctrl Pts',(-0.861652925570091,-0.144299303100741,
-0.721590372101268));
#19394=CARTESIAN_POINT('Ctrl Pts',(-0.848766861100456,-0.0928409665394229,
-0.736604687327351));
#19395=CARTESIAN_POINT('Ctrl Pts',(-0.84559647055299,-0.0762225747374255,
-0.740223768851063));
#19396=CARTESIAN_POINT('Ctrl Pts',(-0.843383895613249,-0.0595300000000001,
-0.742736168477219));
#19397=CARTESIAN_POINT('',(-0.536443649899847,-0.05953,-0.987512846410683));
#19398=CARTESIAN_POINT('Origin',(0.,-0.05953,0.));
#19399=CARTESIAN_POINT('',(0.0548532617164172,-0.05953,-1.12247250791415));
#19400=CARTESIAN_POINT('Ctrl Pts',(-0.536443649899848,-0.0595300000000001,
-0.987512846410683));
#19401=CARTESIAN_POINT('Ctrl Pts',(-0.533501897135712,-0.0762225747374254,
-0.989110885965947));
#19402=CARTESIAN_POINT('Ctrl Pts',(-0.529268075276156,-0.0928409665394227,
-0.991396466802469));
#19403=CARTESIAN_POINT('Ctrl Pts',(-0.511762781179147,-0.144299303100741,
-1.00061845128527));
#19404=CARTESIAN_POINT('Ctrl Pts',(-0.493462957200432,-0.177024326825049,
-1.0099536580922));
#19405=CARTESIAN_POINT('Ctrl Pts',(-0.45280897844858,-0.227269801620063,
-1.02876878445619));
#19406=CARTESIAN_POINT('Ctrl Pts',(-0.425554672694337,-0.251265615809407,
-1.04048957871266));
#19407=CARTESIAN_POINT('Ctrl Pts',(-0.3787731215897,-0.279889827963178,
-1.05829506364875));
#19408=CARTESIAN_POINT('Ctrl Pts',(-0.354166711873529,-0.290879136862659,
-1.06688848765783));
#19409=CARTESIAN_POINT('Ctrl Pts',(-0.302426893214944,-0.305251990234488,
-1.08269251410343));
#19410=CARTESIAN_POINT('Ctrl Pts',(-0.275287440920027,-0.308638795020976,
-1.0898803575765));
#19411=CARTESIAN_POINT('Ctrl Pts',(-0.224855950742601,-0.308638795020976,
-1.10139101611326));
#19412=CARTESIAN_POINT('Ctrl Pts',(-0.19728546073067,-0.305251990234488,
-1.10669035995599));
#19413=CARTESIAN_POINT('Ctrl Pts',(-0.143812384801039,-0.290879136862659,
-1.11490049012186));
#19414=CARTESIAN_POINT('Ctrl Pts',(-0.117914228755037,-0.279889827963178,
-1.1178344036749));
#19415=CARTESIAN_POINT('Ctrl Pts',(-0.0680399972366989,-0.251265615809407,
-1.12208997038458));
#19416=CARTESIAN_POINT('Ctrl Pts',(-0.0383992541984084,-0.227269801620063,
-1.12335509974011));
#19417=CARTESIAN_POINT('Ctrl Pts',(0.00639229239215326,-0.177024326825049,
-1.12404235695137));
#19418=CARTESIAN_POINT('Ctrl Pts',(0.0269302585198977,-0.144299303100741,
-1.12357162229597));
#19419=CARTESIAN_POINT('Ctrl Pts',(0.04670325263426,-0.0928409665394228,
-1.12285816383385));
#19420=CARTESIAN_POINT('Ctrl Pts',(0.0515094706813703,-0.0762225747374255,
-1.12263591311425));
#19421=CARTESIAN_POINT('Ctrl Pts',(0.0548532617164176,-0.0595300000000001,
-1.12247250791414));
#19422=CARTESIAN_POINT('',(0.437601487681057,-0.05953,-1.03511272300331));
#19423=CARTESIAN_POINT('Origin',(0.,-0.05953,0.));
#19424=CARTESIAN_POINT('',(0.911784794170997,-0.05953,-0.656964154625313));
#19425=CARTESIAN_POINT('Ctrl Pts',(0.437601487681056,-0.0595300000000001,
-1.03511272300331));
#19426=CARTESIAN_POINT('Ctrl Pts',(0.440685038163619,-0.0762225747374255,
-1.03380912944435));
#19427=CARTESIAN_POINT('Ctrl Pts',(0.445111721969657,-0.0928409665394228,
-1.03192403056628));
#19428=CARTESIAN_POINT('Ctrl Pts',(0.463236132117164,-0.144299303100741,
-1.0239876538093));
#19429=CARTESIAN_POINT('Ctrl Pts',(0.481944444320713,-0.177024326825049,
-1.01550068154148));
#19430=CARTESIAN_POINT('Ctrl Pts',(0.522002043615455,-0.227269801620064,
-0.995447160474328));
#19431=CARTESIAN_POINT('Ctrl Pts',(0.548158511259203,-0.251265615809407,
-0.981446681891443));
#19432=CARTESIAN_POINT('Ctrl Pts',(0.591247219971725,-0.279889827963178,
-0.955972930713954));
#19433=CARTESIAN_POINT('Ctrl Pts',(0.613307674922609,-0.290879136862659,
-0.942092777160053));
#19434=CARTESIAN_POINT('Ctrl Pts',(0.657923009631182,-0.305251990234487,
-0.91149460735272));
#19435=CARTESIAN_POINT('Ctrl Pts',(0.680463863683393,-0.308638795020976,
-0.894757676234429));
#19436=CARTESIAN_POINT('Ctrl Pts',(0.720906778729542,-0.308638795020976,
-0.862505527716294));
#19437=CARTESIAN_POINT('Ctrl Pts',(0.742239891936899,-0.305251990234488,
-0.844254137480381));
#19438=CARTESIAN_POINT('Ctrl Pts',(0.781998747691872,-0.290879136862659,
-0.80756613568454));
#19439=CARTESIAN_POINT('Ctrl Pts',(0.800439809856112,-0.279889827963178,
-0.789147407129765));
#19440=CARTESIAN_POINT('Ctrl Pts',(0.834863020612702,-0.251265615809407,
-0.752807465209441));
#19441=CARTESIAN_POINT('Ctrl Pts',(0.854332839576145,-0.227269801620064,
-0.73042219438957));
#19442=CARTESIAN_POINT('Ctrl Pts',(0.882797231409153,-0.177024326825049,
-0.695831250979106));
#19443=CARTESIAN_POINT('Ctrl Pts',(0.895234408667242,-0.144299303100741,
-0.679480524217551));
#19444=CARTESIAN_POINT('Ctrl Pts',(0.907004864562642,-0.0928409665394228,
-0.663576540841106));
#19445=CARTESIAN_POINT('Ctrl Pts',(0.909827729890942,-0.0762225747374256,
-0.659680317203144));
#19446=CARTESIAN_POINT('Ctrl Pts',(0.911784794170998,-0.0595300000000001,
-0.656964154625312));
#19447=CARTESIAN_POINT('',(1.08212377959455,-0.05953,-0.303251606722892));
#19448=CARTESIAN_POINT('Origin',(0.,-0.05953,0.));
#19449=CARTESIAN_POINT('',(1.08212377959455,-0.05953,0.303251606722892));
#19450=CARTESIAN_POINT('Ctrl Pts',(1.08212377959455,-0.0595300000000001,
-0.303251606722892));
#19451=CARTESIAN_POINT('Ctrl Pts',(1.0830271513892,-0.0762225747374255,
-0.300028012588062));
#19452=CARTESIAN_POINT('Ctrl Pts',(1.08431331394788,-0.0928409665394228,
-0.2953917518996));
#19453=CARTESIAN_POINT('Ctrl Pts',(1.08940878963422,-0.144299303100741,
-0.276273267473431));
#19454=CARTESIAN_POINT('Ctrl Pts',(1.09443784939331,-0.177024326825049,
-0.256354979351213));
#19455=CARTESIAN_POINT('Ctrl Pts',(1.10373487993589,-0.227269801620064,
-0.212533521233765));
#19456=CARTESIAN_POINT('Ctrl Pts',(1.10909715583869,-0.251265615809407,
-0.183354415742157));
#19457=CARTESIAN_POINT('Ctrl Pts',(1.1160463456491,-0.279889827963178,-0.133783682657561));
#19458=CARTESIAN_POINT('Ctrl Pts',(1.11894887330541,-0.290879136862659,
-0.107881990270302));
#19459=CARTESIAN_POINT('Ctrl Pts',(1.12284346704144,-0.305251990234488,
-0.0539226701638766));
#19460=CARTESIAN_POINT('Ctrl Pts',(1.123812,-0.308638795020976,-0.025864214957475));
#19461=CARTESIAN_POINT('Ctrl Pts',(1.123812,-0.308638795020976,0.025864214957475));
#19462=CARTESIAN_POINT('Ctrl Pts',(1.12284346704144,-0.305251990234488,
0.0539226701638766));
#19463=CARTESIAN_POINT('Ctrl Pts',(1.11894887330541,-0.290879136862659,
0.107881990270302));
#19464=CARTESIAN_POINT('Ctrl Pts',(1.1160463456491,-0.279889827963178,0.133783682657561));
#19465=CARTESIAN_POINT('Ctrl Pts',(1.10909715583869,-0.251265615809407,
0.183354415742157));
#19466=CARTESIAN_POINT('Ctrl Pts',(1.10373487993589,-0.227269801620064,
0.212533521233765));
#19467=CARTESIAN_POINT('Ctrl Pts',(1.09443784939331,-0.177024326825049,
0.256354979351213));
#19468=CARTESIAN_POINT('Ctrl Pts',(1.08940878963422,-0.144299303100741,
0.276273267473431));
#19469=CARTESIAN_POINT('Ctrl Pts',(1.08431331394788,-0.0928409665394228,
0.2953917518996));
#19470=CARTESIAN_POINT('Ctrl Pts',(1.0830271513892,-0.0762225747374255,
0.300028012588062));
#19471=CARTESIAN_POINT('Ctrl Pts',(1.08212377959455,-0.0595300000000001,
0.303251606722892));
#19472=CARTESIAN_POINT('Origin',(0.,-0.05953,0.));
#19473=CARTESIAN_POINT('Origin',(0.,-0.05953,0.));
#19474=CARTESIAN_POINT('',(0.0589974094846122,-0.05953,1.07456964270265));
#19475=CARTESIAN_POINT('Origin',(0.,-0.05953,0.));
#19476=CARTESIAN_POINT('Origin',(-0.244773027351946,-0.05953,1.07242070340001));
#19477=CARTESIAN_POINT('Origin',(-0.244773027351946,0.,1.07242070340001));
#19478=CARTESIAN_POINT('',(-0.519393123750572,-0.05953,0.942555777842682));
#19479=CARTESIAN_POINT('Ctrl Pts',(-0.519393123750572,-0.05953,0.942555777842682));
#19480=CARTESIAN_POINT('Ctrl Pts',(-0.513714466572041,-0.0925528133349865,
0.945684988399766));
#19481=CARTESIAN_POINT('Ctrl Pts',(-0.503136848051455,-0.124911173756694,
0.951483858396181));
#19482=CARTESIAN_POINT('Ctrl Pts',(-0.47593627990192,-0.177924977804098,
0.965323333309091));
#19483=CARTESIAN_POINT('Ctrl Pts',(-0.460931856495794,-0.199697230012983,
0.972669835243841));
#19484=CARTESIAN_POINT('Ctrl Pts',(-0.426157505475872,-0.237895043532788,
0.988400002689705));
#19485=CARTESIAN_POINT('Ctrl Pts',(-0.406380688682952,-0.254319232363049,
0.996771768218699));
#19486=CARTESIAN_POINT('Ctrl Pts',(-0.364750145543744,-0.28018331644634,
1.01272583306292));
#19487=CARTESIAN_POINT('Ctrl Pts',(-0.340838910881557,-0.29104845371857,
1.02112815447116));
#19488=CARTESIAN_POINT('Ctrl Pts',(-0.290495481564827,-0.30527573347708,
1.036574285215));
#19489=CARTESIAN_POINT('Ctrl Pts',(-0.264056468041074,-0.308638795020976,
1.04359501395068));
#19490=CARTESIAN_POINT('Ctrl Pts',(-0.214892249704082,-0.308638795020976,
1.05481642595959));
#19491=CARTESIAN_POINT('Ctrl Pts',(-0.188025341585962,-0.30527573347708,
1.05996242598502));
#19492=CARTESIAN_POINT('Ctrl Pts',(-0.135965654106109,-0.29104845371857,
1.06788913840721));
#19493=CARTESIAN_POINT('Ctrl Pts',(-0.110776745452494,-0.28018331644634,
1.07069360430242));
#19494=CARTESIAN_POINT('Ctrl Pts',(-0.0663467128214646,-0.254319232363049,
1.07438230428002));
#19495=CARTESIAN_POINT('Ctrl Pts',(-0.0448960436540983,-0.237895043532788,
1.07542044338697));
#19496=CARTESIAN_POINT('Ctrl Pts',(-0.00674037211528124,-0.199697230012983,
1.07633607767727));
#19497=CARTESIAN_POINT('Ctrl Pts',(0.00996567398334777,-0.177924977804098,
1.07622728347683));
#19498=CARTESIAN_POINT('Ctrl Pts',(0.0404772621979741,-0.124911173756694,
1.07556023164702));
#19499=CARTESIAN_POINT('Ctrl Pts',(0.0525234025782719,-0.0925528133349865,
1.07492508698591));
#19500=CARTESIAN_POINT('Ctrl Pts',(0.0589974094846124,-0.05953,1.07456964270265));
#19501=CARTESIAN_POINT('Origin',(-0.244773027351946,-0.05953,1.07242070340001));
#19502=CARTESIAN_POINT('Origin',(0.,-0.05953,0.));
#19503=CARTESIAN_POINT('',(-0.803348093619616,-0.05953,0.716109245731214));
#19504=CARTESIAN_POINT('Origin',(0.,-0.05953,0.));
#19505=CARTESIAN_POINT('Origin',(-0.991065754692661,-0.05953,0.477272113029314));
#19506=CARTESIAN_POINT('Origin',(-0.991065754692661,0.,0.477272113029314));
#19507=CARTESIAN_POINT('',(-1.06075609691358,-0.05953,0.181596019242328));
#19508=CARTESIAN_POINT('Ctrl Pts',(-1.06075609691358,-0.05953,0.181596019242328));
#19509=CARTESIAN_POINT('Ctrl Pts',(-1.05966202740332,-0.0925528133349865,
0.187986803072856));
#19510=CARTESIAN_POINT('Ctrl Pts',(-1.05760072925372,-0.124911173756694,
0.199872254546857));
#19511=CARTESIAN_POINT('Ctrl Pts',(-1.05146158959546,-0.177924977804098,
0.22976728653846));
#19512=CARTESIAN_POINT('Ctrl Pts',(-1.04785021111757,-0.199697230012983,
0.246078686169301));
#19513=CARTESIAN_POINT('Ctrl Pts',(-1.03846709802406,-0.237895043532788,
0.283073967563097));
#19514=CARTESIAN_POINT('Ctrl Pts',(-1.03268176429485,-0.254319232363049,
0.303755815985685));
#19515=CARTESIAN_POINT('Ctrl Pts',(-1.01919893537026,-0.28018331644634,
0.346251081972725));
#19516=CARTESIAN_POINT('Ctrl Pts',(-1.01085972381132,-0.29104845371857,
0.370184399726282));
#19517=CARTESIAN_POINT('Ctrl Pts',(-0.99154738033959,-0.30527573347708,
0.419174982698463));
#19518=CARTESIAN_POINT('Ctrl Pts',(-0.980551951791748,-0.308638795020976,
0.444223188605045));
#19519=CARTESIAN_POINT('Ctrl Pts',(-0.958671816228589,-0.308638795020976,
0.489657758261848));
#19520=CARTESIAN_POINT('Ctrl Pts',(-0.945943877838127,-0.30527573347708,
0.51387163140139));
#19521=CARTESIAN_POINT('Ctrl Pts',(-0.91968254693063,-0.29104845371857,
0.559515758398093));
#19522=CARTESIAN_POINT('Ctrl Pts',(-0.906170138993533,-0.28018331644634,
0.580957796077825));
#19523=CARTESIAN_POINT('Ctrl Pts',(-0.8813524085237,-0.254319232363049,
0.617994461173994));
#19524=CARTESIAN_POINT('Ctrl Pts',(-0.868789784891799,-0.237895043532788,
0.635412538795143));
#19525=CARTESIAN_POINT('Ctrl Pts',(-0.845715984518854,-0.199697230012983,
0.66581473268113));
#19526=CARTESIAN_POINT('Ctrl Pts',(-0.835214876415962,-0.177924977804098,
0.678808213394124));
#19527=CARTESIAN_POINT('Ctrl Pts',(-0.815669690204649,-0.124911173756694,
0.702247233627224));
#19528=CARTESIAN_POINT('Ctrl Pts',(-0.807662468433796,-0.0925528133349865,
0.711269279199861));
#19529=CARTESIAN_POINT('Ctrl Pts',(-0.803348093619616,-0.05953,0.716109245731214));
#19530=CARTESIAN_POINT('Origin',(-0.991065754692661,-0.05953,0.477272113029314));
#19531=CARTESIAN_POINT('Origin',(0.,-0.05953,0.));
#19532=CARTESIAN_POINT('',(-1.076188,-0.05953,1.31795018948079E-16));
#19533=CARTESIAN_POINT('Origin',(0.,-0.05953,0.));
#19534=CARTESIAN_POINT('',(-1.06075609691358,-0.05953,-0.181596019242328));
#19535=CARTESIAN_POINT('Origin',(0.,-0.05953,0.));
#19536=CARTESIAN_POINT('Origin',(-0.991065754692661,-0.05953,-0.477272113029314));
#19537=CARTESIAN_POINT('Origin',(-0.991065754692661,0.,-0.477272113029314));
#19538=CARTESIAN_POINT('',(-0.803348093619616,-0.05953,-0.716109245731215));
#19539=CARTESIAN_POINT('Ctrl Pts',(-0.803348093619616,-0.05953,-0.716109245731215));
#19540=CARTESIAN_POINT('Ctrl Pts',(-0.807662468433795,-0.0925528133349865,
-0.711269279199862));
#19541=CARTESIAN_POINT('Ctrl Pts',(-0.815669690204649,-0.124911173756694,
-0.702247233627224));
#19542=CARTESIAN_POINT('Ctrl Pts',(-0.835214876415962,-0.177924977804098,
-0.678808213394124));
#19543=CARTESIAN_POINT('Ctrl Pts',(-0.845715984518854,-0.199697230012983,
-0.66581473268113));
#19544=CARTESIAN_POINT('Ctrl Pts',(-0.868789784891799,-0.237895043532788,
-0.635412538795143));
#19545=CARTESIAN_POINT('Ctrl Pts',(-0.8813524085237,-0.254319232363049,
-0.617994461173994));
#19546=CARTESIAN_POINT('Ctrl Pts',(-0.906170138993533,-0.28018331644634,
-0.580957796077826));
#19547=CARTESIAN_POINT('Ctrl Pts',(-0.91968254693063,-0.29104845371857,
-0.559515758398093));
#19548=CARTESIAN_POINT('Ctrl Pts',(-0.945943877838127,-0.30527573347708,
-0.51387163140139));
#19549=CARTESIAN_POINT('Ctrl Pts',(-0.958671816228589,-0.308638795020976,
-0.489657758261848));
#19550=CARTESIAN_POINT('Ctrl Pts',(-0.980551951791748,-0.308638795020976,
-0.444223188605045));
#19551=CARTESIAN_POINT('Ctrl Pts',(-0.99154738033959,-0.30527573347708,
-0.419174982698463));
#19552=CARTESIAN_POINT('Ctrl Pts',(-1.01085972381132,-0.29104845371857,
-0.370184399726282));
#19553=CARTESIAN_POINT('Ctrl Pts',(-1.01919893537026,-0.28018331644634,
-0.346251081972725));
#19554=CARTESIAN_POINT('Ctrl Pts',(-1.03268176429485,-0.254319232363049,
-0.303755815985685));
#19555=CARTESIAN_POINT('Ctrl Pts',(-1.03846709802406,-0.237895043532788,
-0.283073967563097));
#19556=CARTESIAN_POINT('Ctrl Pts',(-1.04785021111757,-0.199697230012983,
-0.246078686169302));
#19557=CARTESIAN_POINT('Ctrl Pts',(-1.05146158959546,-0.177924977804098,
-0.229767286538461));
#19558=CARTESIAN_POINT('Ctrl Pts',(-1.05760072925372,-0.124911173756694,
-0.199872254546858));
#19559=CARTESIAN_POINT('Ctrl Pts',(-1.05966202740332,-0.0925528133349864,
-0.187986803072857));
#19560=CARTESIAN_POINT('Ctrl Pts',(-1.06075609691358,-0.05953,-0.181596019242328));
#19561=CARTESIAN_POINT('Origin',(-0.991065754692661,-0.05953,-0.477272113029314));
#19562=CARTESIAN_POINT('Origin',(0.,-0.05953,0.));
#19563=CARTESIAN_POINT('',(-0.519393123750572,-0.05953,-0.942555777842682));
#19564=CARTESIAN_POINT('Origin',(0.,-0.05953,0.));
#19565=CARTESIAN_POINT('Origin',(-0.244773027351946,-0.05953,-1.07242070340001));
#19566=CARTESIAN_POINT('Origin',(-0.244773027351946,0.,-1.07242070340001));
#19567=CARTESIAN_POINT('',(0.0589974094846125,-0.05953,-1.07456964270265));
#19568=CARTESIAN_POINT('Ctrl Pts',(0.0589974094846127,-0.05953,-1.07456964270265));
#19569=CARTESIAN_POINT('Ctrl Pts',(0.0525234025782722,-0.0925528133349865,
-1.07492508698591));
#19570=CARTESIAN_POINT('Ctrl Pts',(0.0404772621979744,-0.124911173756694,
-1.07556023164702));
#19571=CARTESIAN_POINT('Ctrl Pts',(0.0099656739833481,-0.177924977804098,
-1.07622728347683));
#19572=CARTESIAN_POINT('Ctrl Pts',(-0.00674037211528096,-0.199697230012983,
-1.07633607767727));
#19573=CARTESIAN_POINT('Ctrl Pts',(-0.044896043654098,-0.237895043532788,
-1.07542044338697));
#19574=CARTESIAN_POINT('Ctrl Pts',(-0.0663467128214644,-0.254319232363049,
-1.07438230428002));
#19575=CARTESIAN_POINT('Ctrl Pts',(-0.110776745452493,-0.28018331644634,
-1.07069360430242));
#19576=CARTESIAN_POINT('Ctrl Pts',(-0.135965654106109,-0.29104845371857,
-1.06788913840721));
#19577=CARTESIAN_POINT('Ctrl Pts',(-0.188025341585962,-0.30527573347708,
-1.05996242598502));
#19578=CARTESIAN_POINT('Ctrl Pts',(-0.214892249704082,-0.308638795020976,
-1.05481642595959));
#19579=CARTESIAN_POINT('Ctrl Pts',(-0.264056468041074,-0.308638795020976,
-1.04359501395068));
#19580=CARTESIAN_POINT('Ctrl Pts',(-0.290495481564827,-0.30527573347708,
-1.036574285215));
#19581=CARTESIAN_POINT('Ctrl Pts',(-0.340838910881557,-0.291048453718569,
-1.02112815447116));
#19582=CARTESIAN_POINT('Ctrl Pts',(-0.364750145543744,-0.28018331644634,
-1.01272583306292));
#19583=CARTESIAN_POINT('Ctrl Pts',(-0.406380688682952,-0.254319232363049,
-0.996771768218699));
#19584=CARTESIAN_POINT('Ctrl Pts',(-0.426157505475872,-0.237895043532788,
-0.988400002689705));
#19585=CARTESIAN_POINT('Ctrl Pts',(-0.460931856495794,-0.199697230012983,
-0.972669835243841));
#19586=CARTESIAN_POINT('Ctrl Pts',(-0.475936279901919,-0.177924977804098,
-0.965323333309091));
#19587=CARTESIAN_POINT('Ctrl Pts',(-0.503136848051454,-0.124911173756694,
-0.951483858396181));
#19588=CARTESIAN_POINT('Ctrl Pts',(-0.513714466572041,-0.0925528133349865,
-0.945684988399766));
#19589=CARTESIAN_POINT('Ctrl Pts',(-0.519393123750572,-0.05953,-0.942555777842682));
#19590=CARTESIAN_POINT('Origin',(-0.244773027351946,-0.05953,-1.07242070340001));
#19591=CARTESIAN_POINT('Origin',(0.,-0.05953,0.));
#19592=CARTESIAN_POINT('',(0.413083465285518,-0.05953,-0.993751811093549));
#19593=CARTESIAN_POINT('Origin',(0.,-0.05953,0.));
#19594=CARTESIAN_POINT('Origin',(0.685838782044607,-0.05953,-0.860014630714833));
#19595=CARTESIAN_POINT('Origin',(0.685838782044607,0.,-0.860014630714833));
#19596=CARTESIAN_POINT('',(0.876916659919095,-0.05953,-0.623857181492959));
#19597=CARTESIAN_POINT('Ctrl Pts',(0.876916659919095,-0.05953,-0.623857181492958));
#19598=CARTESIAN_POINT('Ctrl Pts',(0.873158080166742,-0.0925528133349865,
-0.62914037979579));
#19599=CARTESIAN_POINT('Ctrl Pts',(0.866144010579847,-0.124911173756694,
-0.638954437806245));
#19600=CARTESIAN_POINT('Ctrl Pts',(0.847641868610495,-0.177924977804098,
-0.663225258065736));
#19601=CARTESIAN_POINT('Ctrl Pts',(0.837310877969633,-0.199697230012983,
-0.676354402927683));
#19602=CARTESIAN_POINT('Ctrl Pts',(0.81280533416753,-0.237895043532788,
-0.705614819529209));
#19603=CARTESIAN_POINT('Ctrl Pts',(0.798619410861634,-0.254319232363049,
-0.721738358858166));
#19604=CARTESIAN_POINT('Ctrl Pts',(0.768033796848072,-0.28018331644634,
-0.754175290318038));
#19605=CARTESIAN_POINT('Ctrl Pts',(0.750136149454208,-0.29104845371857,
-0.772120216227122));
#19606=CARTESIAN_POINT('Ctrl Pts',(0.711480111898423,-0.30527573347708,
-0.807879894508811));
#19607=CARTESIAN_POINT('Ctrl Pts',(0.690705563850638,-0.308638795020976,
-0.825676810575913));
#19608=CARTESIAN_POINT('Ctrl Pts',(0.651278921914856,-0.308638795020976,
-0.857118508332695));
#19609=CARTESIAN_POINT('Ctrl Pts',(0.629305439856167,-0.30527573347708,
-0.873412008702649));
#19610=CARTESIAN_POINT('Ctrl Pts',(0.585840553788742,-0.29104845371857,
-0.903141581680914));
#19611=CARTESIAN_POINT('Ctrl Pts',(0.564362943424239,-0.28018331644634,
-0.916597376014514));
#19612=CARTESIAN_POINT('Ctrl Pts',(0.525933334162556,-0.254319232363049,
-0.939198248544427));
#19613=CARTESIAN_POINT('Ctrl Pts',(0.507057380724533,-0.237895043532788,
-0.949440676105255));
#19614=CARTESIAN_POINT('Ctrl Pts',(0.473077587363686,-0.199697230012983,
-0.966820759530997));
#19615=CARTESIAN_POINT('Ctrl Pts',(0.457978755888596,-0.177924977804098,
-0.973971221090534));
#19616=CARTESIAN_POINT('Ctrl Pts',(0.430199341854858,-0.124911173756694,
-0.986608710139579));
#19617=CARTESIAN_POINT('Ctrl Pts',(0.419070565453384,-0.0925528133349865,
-0.991263089003441));
#19618=CARTESIAN_POINT('Ctrl Pts',(0.413083465285518,-0.05953,-0.993751811093549));
#19619=CARTESIAN_POINT('Origin',(0.685838782044607,-0.05953,-0.860014630714833));
#19620=CARTESIAN_POINT('Origin',(0.,-0.208355,0.));
#19621=CARTESIAN_POINT('',(-1.076188,-0.35718,1.31795018948079E-16));
#19622=CARTESIAN_POINT('Origin',(0.,-0.35718,0.));
#19623=CARTESIAN_POINT('',(-1.076188,-0.208355,1.31795018948079E-16));
#19624=CARTESIAN_POINT('',(1.03449977959455,-0.05953,0.296632461748266));
#19625=CARTESIAN_POINT('Origin',(0.,-0.05953,0.));
#19626=CARTESIAN_POINT('',(1.03449977959455,-0.05953,-0.296632461748266));
#19627=CARTESIAN_POINT('Ctrl Pts',(1.03449977959455,-0.05953,0.296632461748267));
#19628=CARTESIAN_POINT('Ctrl Pts',(1.03628691421076,-0.0925528133349865,
0.290399865505497));
#19629=CARTESIAN_POINT('Ctrl Pts',(1.03958665287714,-0.124911173756694,
0.278797079997872));
#19630=CARTESIAN_POINT('Ctrl Pts',(1.0470264474309,-0.177924977804098,0.249198913998601));
#19631=CARTESIAN_POINT('Ctrl Pts',(1.05084995891418,-0.199697230012983,
0.232935932341942));
#19632=CARTESIAN_POINT('Ctrl Pts',(1.05844771715377,-0.237895043532788,
0.195533155353269));
#19633=CARTESIAN_POINT('Ctrl Pts',(1.06220882929878,-0.254319232363049,
0.17438929156337));
#19634=CARTESIAN_POINT('Ctrl Pts',(1.06849922508772,-0.28018331644634,0.130252399648131));
#19635=CARTESIAN_POINT('Ctrl Pts',(1.07137013248666,-0.29104845371857,0.105070977154072));
#19636=CARTESIAN_POINT('Ctrl Pts',(1.07522652957392,-0.30527573347708,0.0525526752791107));
#19637=CARTESIAN_POINT('Ctrl Pts',(1.076188,-0.308638795020976,0.025214283908933));
#19638=CARTESIAN_POINT('Ctrl Pts',(1.076188,-0.308638795020976,-0.025214283908933));
#19639=CARTESIAN_POINT('Ctrl Pts',(1.07522652957392,-0.30527573347708,-0.0525526752791107));
#19640=CARTESIAN_POINT('Ctrl Pts',(1.07137013248666,-0.29104845371857,-0.105070977154072));
#19641=CARTESIAN_POINT('Ctrl Pts',(1.06849922508772,-0.28018331644634,-0.130252399648131));
#19642=CARTESIAN_POINT('Ctrl Pts',(1.06220882929878,-0.254319232363049,
-0.17438929156337));
#19643=CARTESIAN_POINT('Ctrl Pts',(1.05844771715377,-0.237895043532788,
-0.195533155353269));
#19644=CARTESIAN_POINT('Ctrl Pts',(1.05084995891418,-0.199697230012983,
-0.232935932341942));
#19645=CARTESIAN_POINT('Ctrl Pts',(1.0470264474309,-0.177924977804098,-0.249198913998601));
#19646=CARTESIAN_POINT('Ctrl Pts',(1.03958665287714,-0.124911173756694,
-0.278797079997872));
#19647=CARTESIAN_POINT('Ctrl Pts',(1.03628691421076,-0.0925528133349865,
-0.290399865505497));
#19648=CARTESIAN_POINT('Ctrl Pts',(1.03449977959455,-0.05953,-0.296632461748267));
#19649=CARTESIAN_POINT('Origin',(0.,-0.05953,0.));
#19650=CARTESIAN_POINT('Origin',(0.,-0.05953,0.));
#19651=CARTESIAN_POINT('Origin',(1.1,-0.05953,0.));
#19652=CARTESIAN_POINT('Origin',(1.1,0.,0.));
#19653=CARTESIAN_POINT('Origin',(1.1,-0.05953,0.));
#19654=CARTESIAN_POINT('Origin',(0.,-0.35718,0.));
#19655=CARTESIAN_POINT('Origin',(0.,-0.05953,0.));
#33219=UNCERTAINTY_MEASURE_WITH_UNIT(LENGTH_MEASURE(0.001),#33300,
'DISTANCE_ACCURACY_VALUE',
'Maximum model space distance between geometric entities at asserted c
onnectivities');
#33247=UNCERTAINTY_MEASURE_WITH_UNIT(LENGTH_MEASURE(0.001),#33300,
'DISTANCE_ACCURACY_VALUE',
'Maximum model space distance between geometric entities at asserted c
onnectivities');
#33271=(
GEOMETRIC_REPRESENTATION_CONTEXT(3)
GLOBAL_UNCERTAINTY_ASSIGNED_CONTEXT((#33219))
GLOBAL_UNIT_ASSIGNED_CONTEXT((#33300,#33302,#33303))
REPRESENTATION_CONTEXT('','3D')
);
#33299=(
GEOMETRIC_REPRESENTATION_CONTEXT(3)
GLOBAL_UNCERTAINTY_ASSIGNED_CONTEXT((#33247))
GLOBAL_UNIT_ASSIGNED_CONTEXT((#33300,#33302,#33303))
REPRESENTATION_CONTEXT('','3D')
);
#33300=(
LENGTH_UNIT()
NAMED_UNIT(*)
SI_UNIT(.CENTI.,.METRE.)
);
#33302=(
NAMED_UNIT(*)
PLANE_ANGLE_UNIT()
SI_UNIT($,.RADIAN.)
);
#33303=(
NAMED_UNIT(*)
SI_UNIT($,.STERADIAN.)
SOLID_ANGLE_UNIT()
);
#33327=SHAPE_DEFINITION_REPRESENTATION(#33378,#33509);
#33378=PRODUCT_DEFINITION_SHAPE('',$,#33561);
#33509=SHAPE_REPRESENTATION('',(#13659),#33271);
#33537=PRODUCT_DEFINITION_CONTEXT('part definition',#33692,'design');
#33561=PRODUCT_DEFINITION('Cage','Cage',#33612,#33537);
#33612=PRODUCT_DEFINITION_FORMATION('',$,#33717);
#33692=APPLICATION_CONTEXT(
'Core Data for Automotive Mechanical Design Process');
#33693=PRODUCT_CONTEXT('part definition',#33692,'mechanical');
#33717=PRODUCT('Cage','Cage','Cage',(#33693));
#33808=COLOUR_RGB('Grey',0.48,0.52,0.57);
#33809=FILL_AREA_STYLE_COLOUR('',#33808);
#33810=FILL_AREA_STYLE('',(#33809));
#33811=SURFACE_STYLE_FILL_AREA(#33810);
#33812=SURFACE_SIDE_STYLE('',(#33811));
#33813=SURFACE_STYLE_USAGE(.BOTH.,#33812);
#33814=PRESENTATION_STYLE_ASSIGNMENT((#33813));
ENDSEC;
END-ISO-10303-21;
